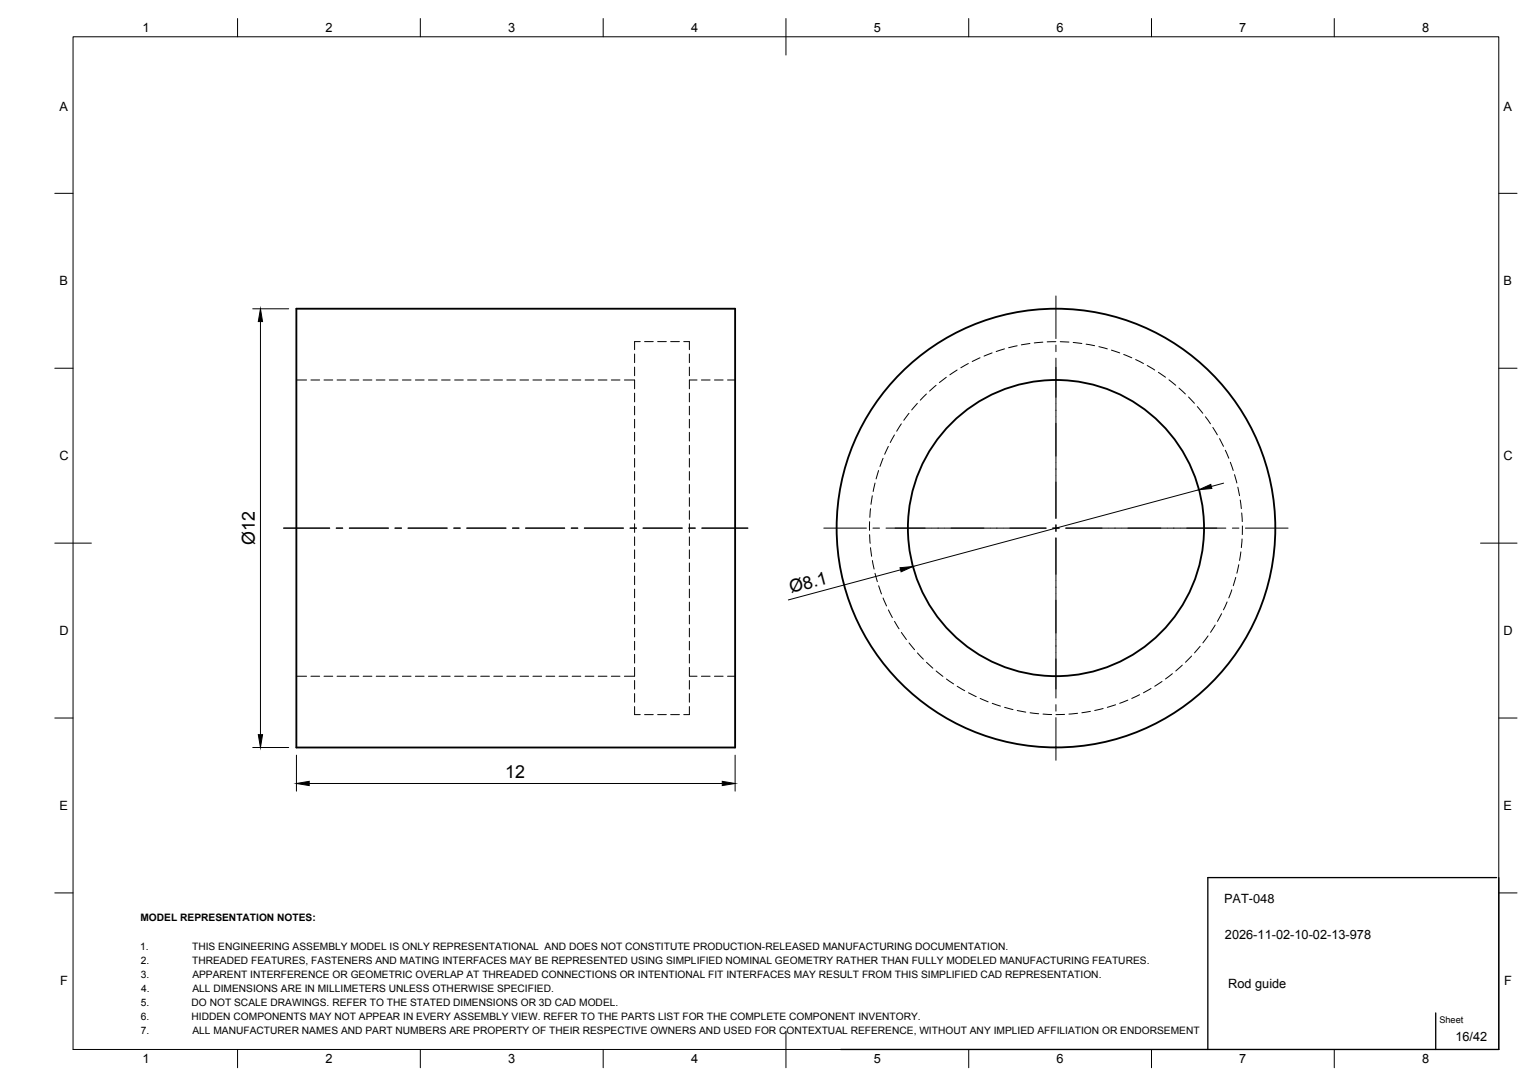
ISO-10303-21;
HEADER;
/* Generated by software containing ST-Developer
 * from STEP Tools, Inc. (www.steptools.com) 
 */

FILE_DESCRIPTION(
/* description */ ('Guided pneumatic stop gate'),
/* implementation_level */ '2;1');

FILE_NAME(
/* name */ 'Rod guide.step',
/* time_stamp */ '2026-10-27T21:43:45-07:00',
/* author */ (''),
/* organization */ (''),
/* preprocessor_version */ 'ST-DEVELOPER v20.2',
/* originating_system */ 'Autodesk Translation Framework v15.17.0.0',
/* authorisation */ '');

FILE_SCHEMA (('AUTOMOTIVE_DESIGN { 1 0 10303 214 3 1 1 }'));
ENDSEC;

DATA;
#10=MECHANICAL_DESIGN_GEOMETRIC_PRESENTATION_REPRESENTATION('',(#549),#14392);
#465=SHAPE_REPRESENTATION_RELATIONSHIP('SRR','None',#14600,#507);
#507=ADVANCED_BREP_SHAPE_REPRESENTATION('',(#590),#14362);
#549=STYLED_ITEM('',(#14891),#590);
#590=MANIFOLD_SOLID_BREP('Body1',#7890);
#691=FACE_BOUND('',#1875,.T.);
#692=FACE_BOUND('',#1877,.T.);
#693=FACE_BOUND('',#1882,.T.);
#694=FACE_BOUND('',#1884,.T.);
#963=PLANE('',#8775);
#964=PLANE('',#8777);
#965=PLANE('',#8786);
#966=PLANE('',#8787);
#1322=FACE_OUTER_BOUND('',#1873,.T.);
#1323=FACE_OUTER_BOUND('',#1874,.T.);
#1324=FACE_OUTER_BOUND('',#1876,.T.);
#1325=FACE_OUTER_BOUND('',#1878,.T.);
#1326=FACE_OUTER_BOUND('',#1879,.T.);
#1327=FACE_OUTER_BOUND('',#1880,.T.);
#1328=FACE_OUTER_BOUND('',#1881,.T.);
#1329=FACE_OUTER_BOUND('',#1883,.T.);
#1873=EDGE_LOOP('',(#6122,#6123,#6124,#6125));
#1874=EDGE_LOOP('',(#6126));
#1875=EDGE_LOOP('',(#6127));
#1876=EDGE_LOOP('',(#6128));
#1877=EDGE_LOOP('',(#6129));
#1878=EDGE_LOOP('',(#6130,#6131,#6132,#6133));
#1879=EDGE_LOOP('',(#6134,#6135,#6136,#6137));
#1880=EDGE_LOOP('',(#6138,#6139,#6140,#6141));
#1881=EDGE_LOOP('',(#6142));
#1882=EDGE_LOOP('',(#6143));
#1883=EDGE_LOOP('',(#6144));
#1884=EDGE_LOOP('',(#6145));
#2517=LINE('',#12806,#3062);
#2518=LINE('',#12816,#3063);
#2519=LINE('',#12821,#3064);
#2520=LINE('',#12826,#3065);
#3062=VECTOR('',#10400,0.51);
#3063=VECTOR('',#10413,0.405);
#3064=VECTOR('',#10420,0.405);
#3065=VECTOR('',#10425,0.6);
#3518=CIRCLE('',#8773,0.51);
#3519=CIRCLE('',#8774,0.51);
#3520=CIRCLE('',#8776,0.405);
#3521=CIRCLE('',#8778,0.405);
#3522=CIRCLE('',#8780,0.405);
#3523=CIRCLE('',#8782,0.405);
#3524=CIRCLE('',#8784,0.6);
#3525=CIRCLE('',#8785,0.6);
#3992=VERTEX_POINT('',#12803);
#3993=VERTEX_POINT('',#12805);
#3994=VERTEX_POINT('',#12809);
#3995=VERTEX_POINT('',#12812);
#3996=VERTEX_POINT('',#12815);
#3997=VERTEX_POINT('',#12819);
#3998=VERTEX_POINT('',#12823);
#3999=VERTEX_POINT('',#12825);
#4759=EDGE_CURVE('',#3992,#3992,#3518,.T.);
#4760=EDGE_CURVE('',#3992,#3993,#2517,.T.);
#4761=EDGE_CURVE('',#3993,#3993,#3519,.T.);
#4762=EDGE_CURVE('',#3994,#3994,#3520,.T.);
#4763=EDGE_CURVE('',#3995,#3995,#3521,.T.);
#4764=EDGE_CURVE('',#3995,#3996,#2518,.T.);
#4765=EDGE_CURVE('',#3996,#3996,#3522,.T.);
#4766=EDGE_CURVE('',#3997,#3997,#3523,.T.);
#4767=EDGE_CURVE('',#3997,#3994,#2519,.T.);
#4768=EDGE_CURVE('',#3998,#3998,#3524,.T.);
#4769=EDGE_CURVE('',#3998,#3999,#2520,.T.);
#4770=EDGE_CURVE('',#3999,#3999,#3525,.T.);
#6122=ORIENTED_EDGE('',*,*,#4759,.F.);
#6123=ORIENTED_EDGE('',*,*,#4760,.T.);
#6124=ORIENTED_EDGE('',*,*,#4761,.T.);
#6125=ORIENTED_EDGE('',*,*,#4760,.F.);
#6126=ORIENTED_EDGE('',*,*,#4761,.F.);
#6127=ORIENTED_EDGE('',*,*,#4762,.F.);
#6128=ORIENTED_EDGE('',*,*,#4759,.T.);
#6129=ORIENTED_EDGE('',*,*,#4763,.F.);
#6130=ORIENTED_EDGE('',*,*,#4763,.T.);
#6131=ORIENTED_EDGE('',*,*,#4764,.T.);
#6132=ORIENTED_EDGE('',*,*,#4765,.T.);
#6133=ORIENTED_EDGE('',*,*,#4764,.F.);
#6134=ORIENTED_EDGE('',*,*,#4766,.F.);
#6135=ORIENTED_EDGE('',*,*,#4767,.T.);
#6136=ORIENTED_EDGE('',*,*,#4762,.T.);
#6137=ORIENTED_EDGE('',*,*,#4767,.F.);
#6138=ORIENTED_EDGE('',*,*,#4768,.F.);
#6139=ORIENTED_EDGE('',*,*,#4769,.T.);
#6140=ORIENTED_EDGE('',*,*,#4770,.T.);
#6141=ORIENTED_EDGE('',*,*,#4769,.F.);
#6142=ORIENTED_EDGE('',*,*,#4768,.T.);
#6143=ORIENTED_EDGE('',*,*,#4766,.T.);
#6144=ORIENTED_EDGE('',*,*,#4770,.F.);
#6145=ORIENTED_EDGE('',*,*,#4765,.F.);
#7307=CYLINDRICAL_SURFACE('',#8772,0.51);
#7308=CYLINDRICAL_SURFACE('',#8779,0.405);
#7309=CYLINDRICAL_SURFACE('',#8781,0.405);
#7310=CYLINDRICAL_SURFACE('',#8783,0.6);
#7604=ADVANCED_FACE('',(#1322),#7307,.F.);
#7605=ADVANCED_FACE('',(#1323,#691),#963,.F.);
#7606=ADVANCED_FACE('',(#1324,#692),#964,.T.);
#7607=ADVANCED_FACE('',(#1325),#7308,.F.);
#7608=ADVANCED_FACE('',(#1326),#7309,.F.);
#7609=ADVANCED_FACE('',(#1327),#7310,.T.);
#7610=ADVANCED_FACE('',(#1328,#693),#965,.T.);
#7611=ADVANCED_FACE('',(#1329,#694),#966,.F.);
#7890=CLOSED_SHELL('',(#7604,#7605,#7606,#7607,#7608,#7609,#7610,#7611));
#8771=AXIS2_PLACEMENT_3D('',#12801,#10394,#10395);
#8772=AXIS2_PLACEMENT_3D('',#12802,#10396,#10397);
#8773=AXIS2_PLACEMENT_3D('',#12804,#10398,#10399);
#8774=AXIS2_PLACEMENT_3D('',#12807,#10401,#10402);
#8775=AXIS2_PLACEMENT_3D('',#12808,#10403,#10404);
#8776=AXIS2_PLACEMENT_3D('',#12810,#10405,#10406);
#8777=AXIS2_PLACEMENT_3D('',#12811,#10407,#10408);
#8778=AXIS2_PLACEMENT_3D('',#12813,#10409,#10410);
#8779=AXIS2_PLACEMENT_3D('',#12814,#10411,#10412);
#8780=AXIS2_PLACEMENT_3D('',#12817,#10414,#10415);
#8781=AXIS2_PLACEMENT_3D('',#12818,#10416,#10417);
#8782=AXIS2_PLACEMENT_3D('',#12820,#10418,#10419);
#8783=AXIS2_PLACEMENT_3D('',#12822,#10421,#10422);
#8784=AXIS2_PLACEMENT_3D('',#12824,#10423,#10424);
#8785=AXIS2_PLACEMENT_3D('',#12827,#10426,#10427);
#8786=AXIS2_PLACEMENT_3D('',#12828,#10428,#10429);
#8787=AXIS2_PLACEMENT_3D('',#12829,#10430,#10431);
#10394=DIRECTION('axis',(0.,0.,1.));
#10395=DIRECTION('refdir',(1.,0.,0.));
#10396=DIRECTION('center_axis',(0.,1.,0.));
#10397=DIRECTION('ref_axis',(1.,0.,0.));
#10398=DIRECTION('center_axis',(0.,1.,0.));
#10399=DIRECTION('ref_axis',(1.,0.,0.));
#10400=DIRECTION('',(0.,1.,0.));
#10401=DIRECTION('center_axis',(0.,1.,0.));
#10402=DIRECTION('ref_axis',(1.,0.,0.));
#10403=DIRECTION('center_axis',(0.,1.,0.));
#10404=DIRECTION('ref_axis',(1.,0.,0.));
#10405=DIRECTION('center_axis',(0.,-1.,0.));
#10406=DIRECTION('ref_axis',(1.,0.,0.));
#10407=DIRECTION('center_axis',(0.,1.,0.));
#10408=DIRECTION('ref_axis',(1.,0.,0.));
#10409=DIRECTION('center_axis',(0.,1.,0.));
#10410=DIRECTION('ref_axis',(1.,0.,0.));
#10411=DIRECTION('center_axis',(0.,1.,0.));
#10412=DIRECTION('ref_axis',(1.,0.,0.));
#10413=DIRECTION('',(0.,-1.,0.));
#10414=DIRECTION('center_axis',(0.,-1.,0.));
#10415=DIRECTION('ref_axis',(1.,0.,0.));
#10416=DIRECTION('center_axis',(0.,1.,0.));
#10417=DIRECTION('ref_axis',(1.,0.,0.));
#10418=DIRECTION('center_axis',(0.,-1.,0.));
#10419=DIRECTION('ref_axis',(1.,0.,0.));
#10420=DIRECTION('',(0.,-1.,0.));
#10421=DIRECTION('center_axis',(0.,1.,0.));
#10422=DIRECTION('ref_axis',(1.,0.,0.));
#10423=DIRECTION('center_axis',(0.,1.,0.));
#10424=DIRECTION('ref_axis',(1.,0.,0.));
#10425=DIRECTION('',(0.,-1.,0.));
#10426=DIRECTION('center_axis',(0.,1.,0.));
#10427=DIRECTION('ref_axis',(1.,0.,0.));
#10428=DIRECTION('center_axis',(0.,1.,0.));
#10429=DIRECTION('ref_axis',(1.,0.,0.));
#10430=DIRECTION('center_axis',(0.,1.,0.));
#10431=DIRECTION('ref_axis',(1.,0.,0.));
#12801=CARTESIAN_POINT('',(0.,0.,0.));
#12802=CARTESIAN_POINT('Origin',(0.,0.125,4.5));
#12803=CARTESIAN_POINT('',(-0.51,0.125,4.5));
#12804=CARTESIAN_POINT('Origin',(0.,0.125,4.5));
#12805=CARTESIAN_POINT('',(-0.51,0.275,4.5));
#12806=CARTESIAN_POINT('',(-0.51,0.125,4.5));
#12807=CARTESIAN_POINT('Origin',(0.,0.275,4.5));
#12808=CARTESIAN_POINT('Origin',(0.,0.275,4.5));
#12809=CARTESIAN_POINT('',(-0.405,0.275,4.5));
#12810=CARTESIAN_POINT('Origin',(0.,0.275,4.5));
#12811=CARTESIAN_POINT('Origin',(0.,0.125,4.5));
#12812=CARTESIAN_POINT('',(-0.405,0.125,4.5));
#12813=CARTESIAN_POINT('Origin',(0.,0.125,4.5));
#12814=CARTESIAN_POINT('Origin',(0.,0.,4.5));
#12815=CARTESIAN_POINT('',(-0.405,0.,4.5));
#12816=CARTESIAN_POINT('',(-0.405,0.,4.5));
#12817=CARTESIAN_POINT('Origin',(0.,0.,4.5));
#12818=CARTESIAN_POINT('Origin',(0.,0.,4.5));
#12819=CARTESIAN_POINT('',(-0.405,1.2,4.5));
#12820=CARTESIAN_POINT('Origin',(0.,1.2,4.5));
#12821=CARTESIAN_POINT('',(-0.405,0.,4.5));
#12822=CARTESIAN_POINT('Origin',(0.,0.,4.5));
#12823=CARTESIAN_POINT('',(-0.6,1.2,4.5));
#12824=CARTESIAN_POINT('Origin',(0.,1.2,4.5));
#12825=CARTESIAN_POINT('',(-0.6,0.,4.5));
#12826=CARTESIAN_POINT('',(-0.6,0.,4.5));
#12827=CARTESIAN_POINT('Origin',(0.,0.,4.5));
#12828=CARTESIAN_POINT('Origin',(0.,1.2,4.5));
#12829=CARTESIAN_POINT('Origin',(0.,0.,4.5));
#14314=UNCERTAINTY_MEASURE_WITH_UNIT(LENGTH_MEASURE(0.001),#14393,
'DISTANCE_ACCURACY_VALUE',
'Maximum model space distance between geometric entities at asserted c
onnectivities');
#14344=UNCERTAINTY_MEASURE_WITH_UNIT(LENGTH_MEASURE(0.001),#14393,
'DISTANCE_ACCURACY_VALUE',
'Maximum model space distance between geometric entities at asserted c
onnectivities');
#14362=(
GEOMETRIC_REPRESENTATION_CONTEXT(3)
GLOBAL_UNCERTAINTY_ASSIGNED_CONTEXT((#14314))
GLOBAL_UNIT_ASSIGNED_CONTEXT((#14393,#14395,#14396))
REPRESENTATION_CONTEXT('','3D')
);
#14392=(
GEOMETRIC_REPRESENTATION_CONTEXT(3)
GLOBAL_UNCERTAINTY_ASSIGNED_CONTEXT((#14344))
GLOBAL_UNIT_ASSIGNED_CONTEXT((#14393,#14395,#14396))
REPRESENTATION_CONTEXT('','3D')
);
#14393=(
LENGTH_UNIT()
NAMED_UNIT(*)
SI_UNIT(.CENTI.,.METRE.)
);
#14395=(
NAMED_UNIT(*)
PLANE_ANGLE_UNIT()
SI_UNIT($,.RADIAN.)
);
#14396=(
NAMED_UNIT(*)
SI_UNIT($,.STERADIAN.)
SOLID_ANGLE_UNIT()
);
#14414=SHAPE_DEFINITION_REPRESENTATION(#14463,#14600);
#14463=PRODUCT_DEFINITION_SHAPE('',$,#14648);
#14600=SHAPE_REPRESENTATION('',(#8771),#14362);
#14630=PRODUCT_DEFINITION_CONTEXT('part definition',#14773,'design');
#14648=PRODUCT_DEFINITION('Rod guide','Rod guide',#14695,#14630);
#14695=PRODUCT_DEFINITION_FORMATION('',$,#14792);
#14773=APPLICATION_CONTEXT(
'Core Data for Automotive Mechanical Design Process');
#14774=PRODUCT_CONTEXT('part definition',#14773,'mechanical');
#14792=PRODUCT('Rod guide','Rod guide','Rod guide',(#14774));
#14885=COLOUR_RGB('Grey',0.48,0.52,0.57);
#14886=FILL_AREA_STYLE_COLOUR('',#14885);
#14887=FILL_AREA_STYLE('',(#14886));
#14888=SURFACE_STYLE_FILL_AREA(#14887);
#14889=SURFACE_SIDE_STYLE('',(#14888));
#14890=SURFACE_STYLE_USAGE(.BOTH.,#14889);
#14891=PRESENTATION_STYLE_ASSIGNMENT((#14890));
ENDSEC;
END-ISO-10303-21;
